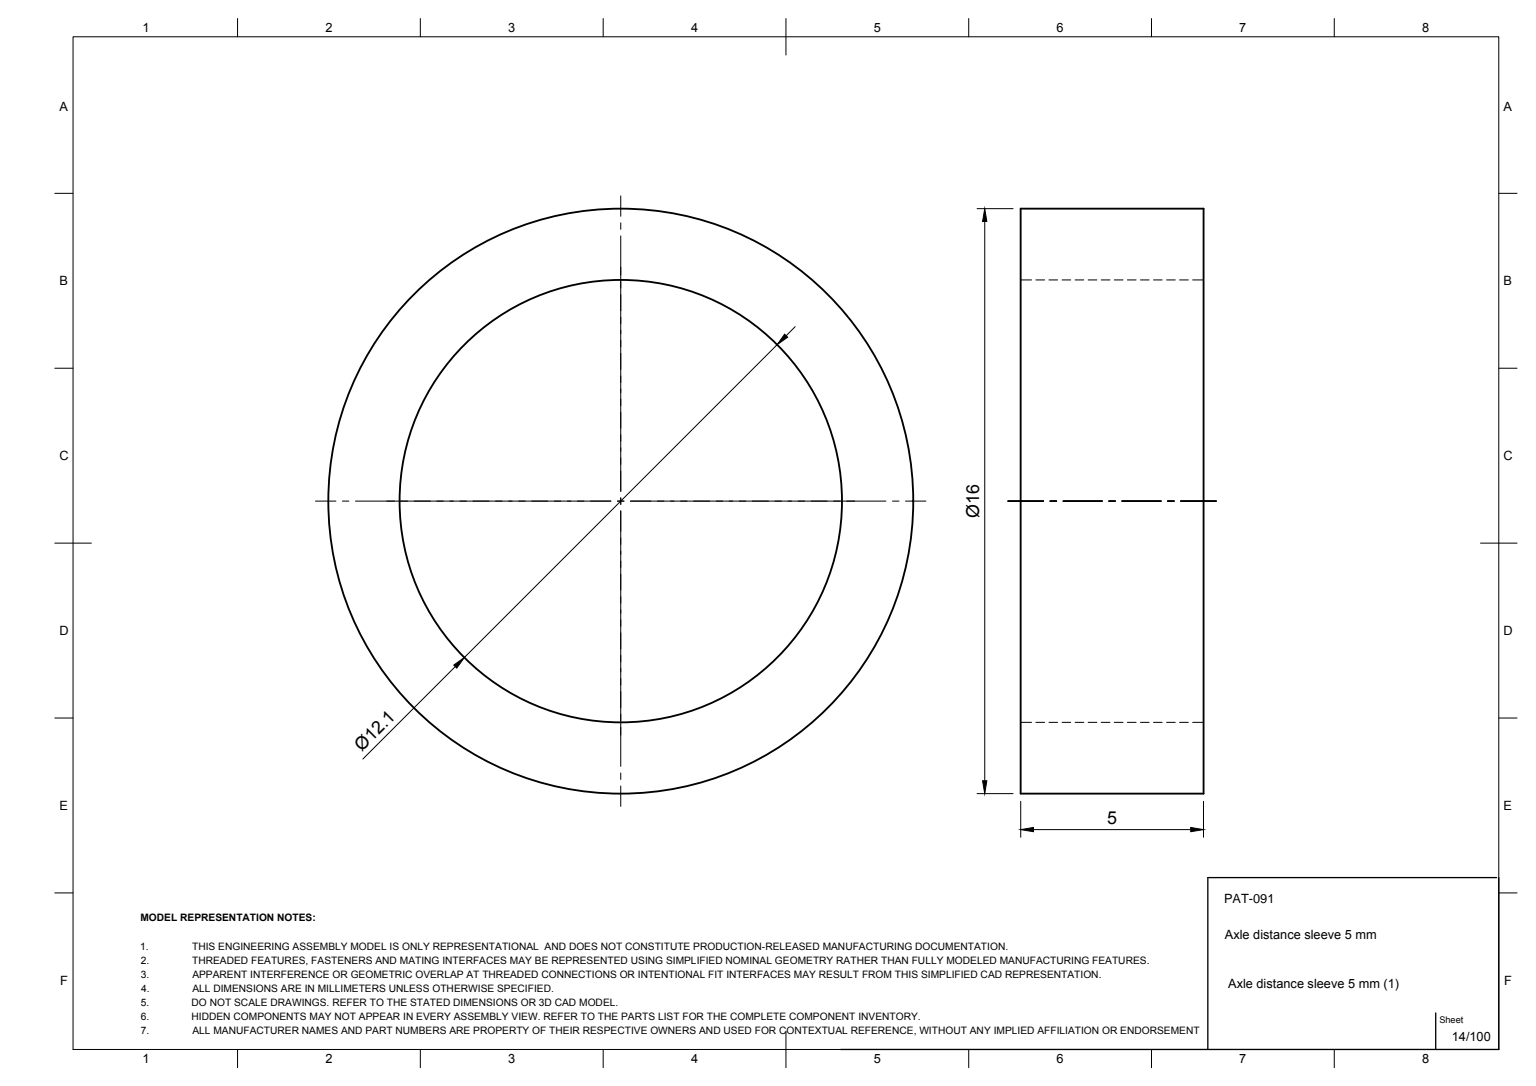
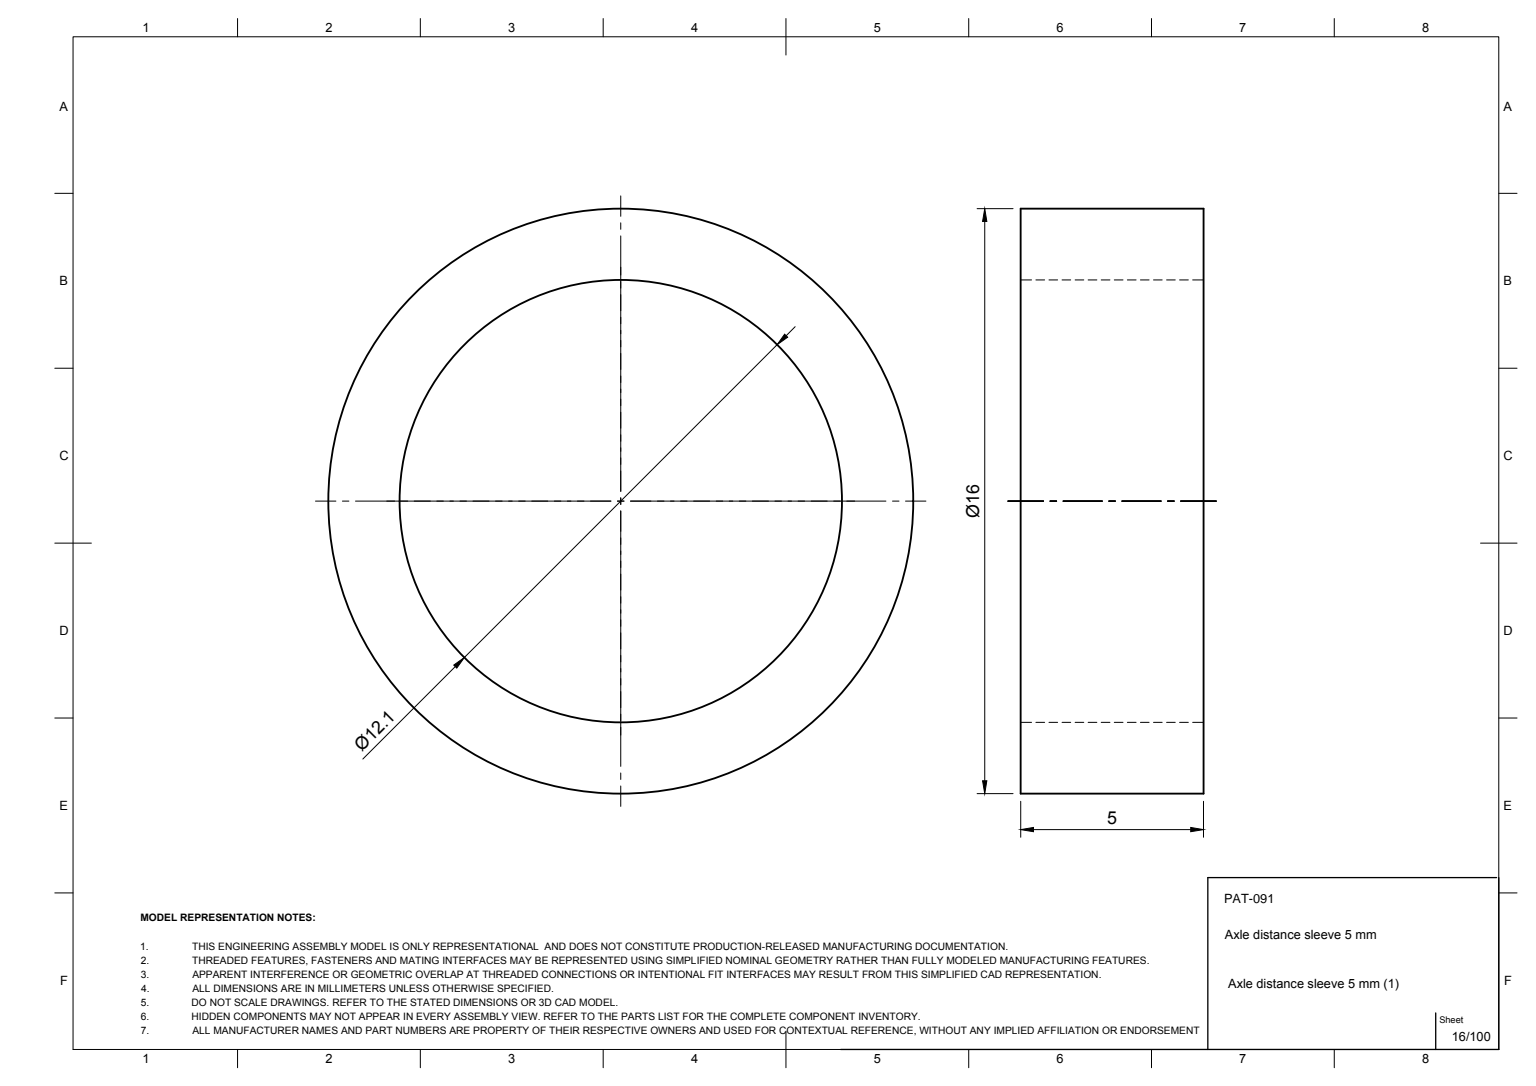
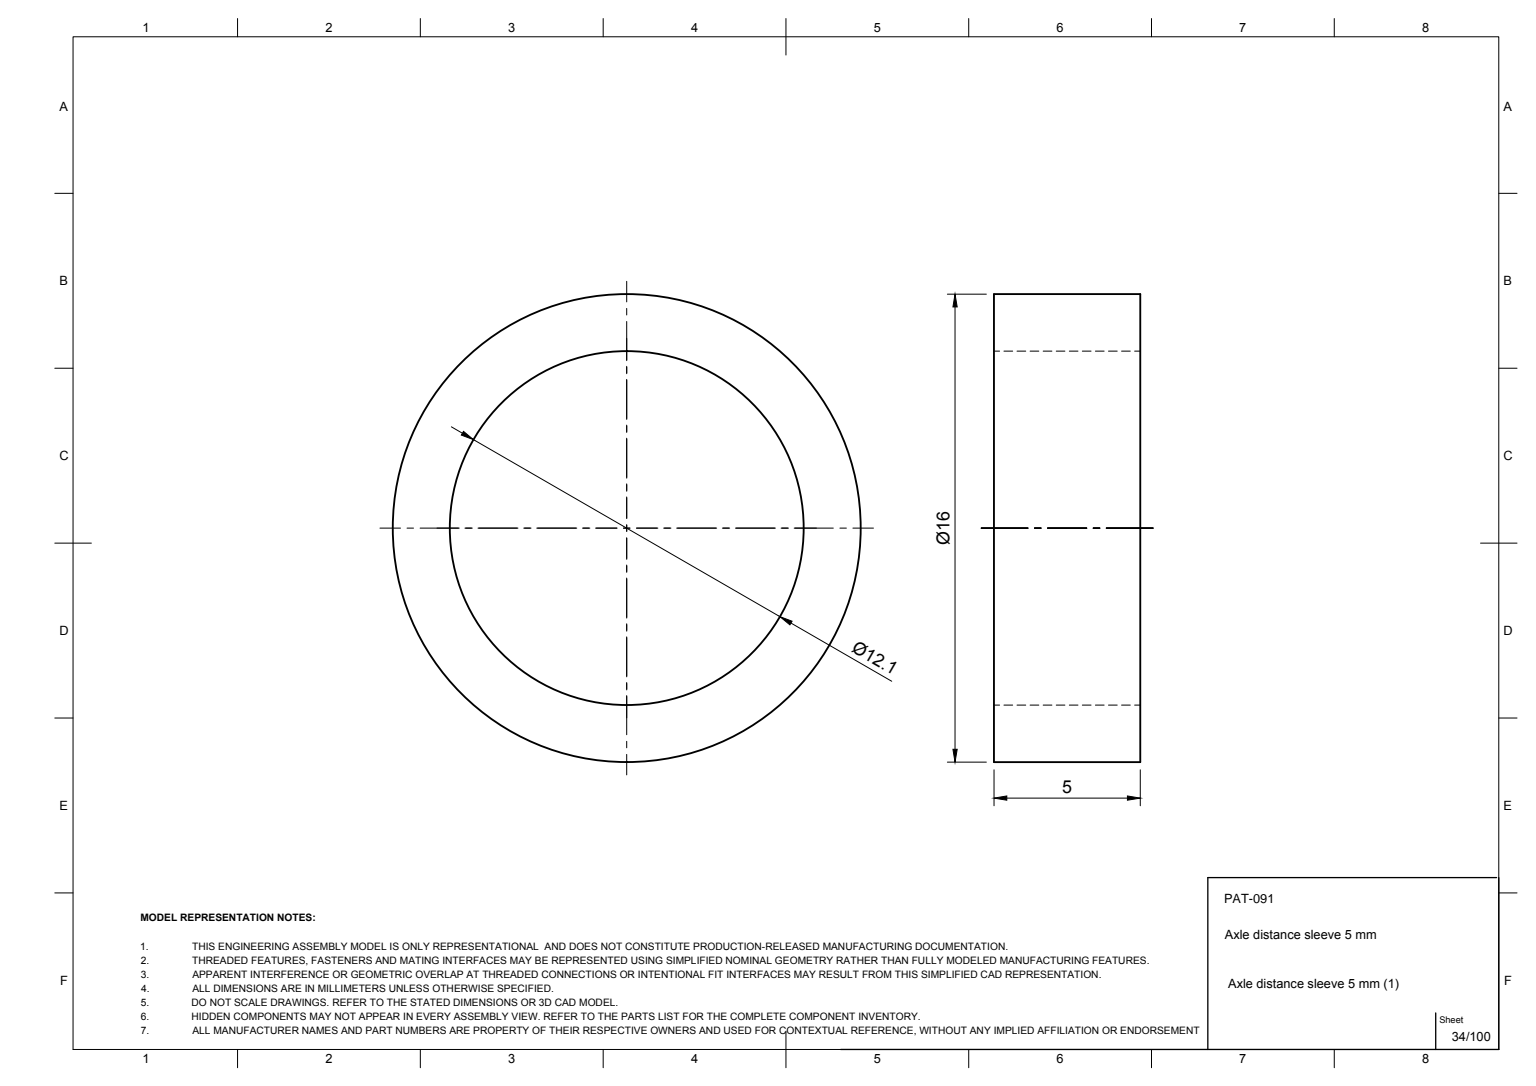
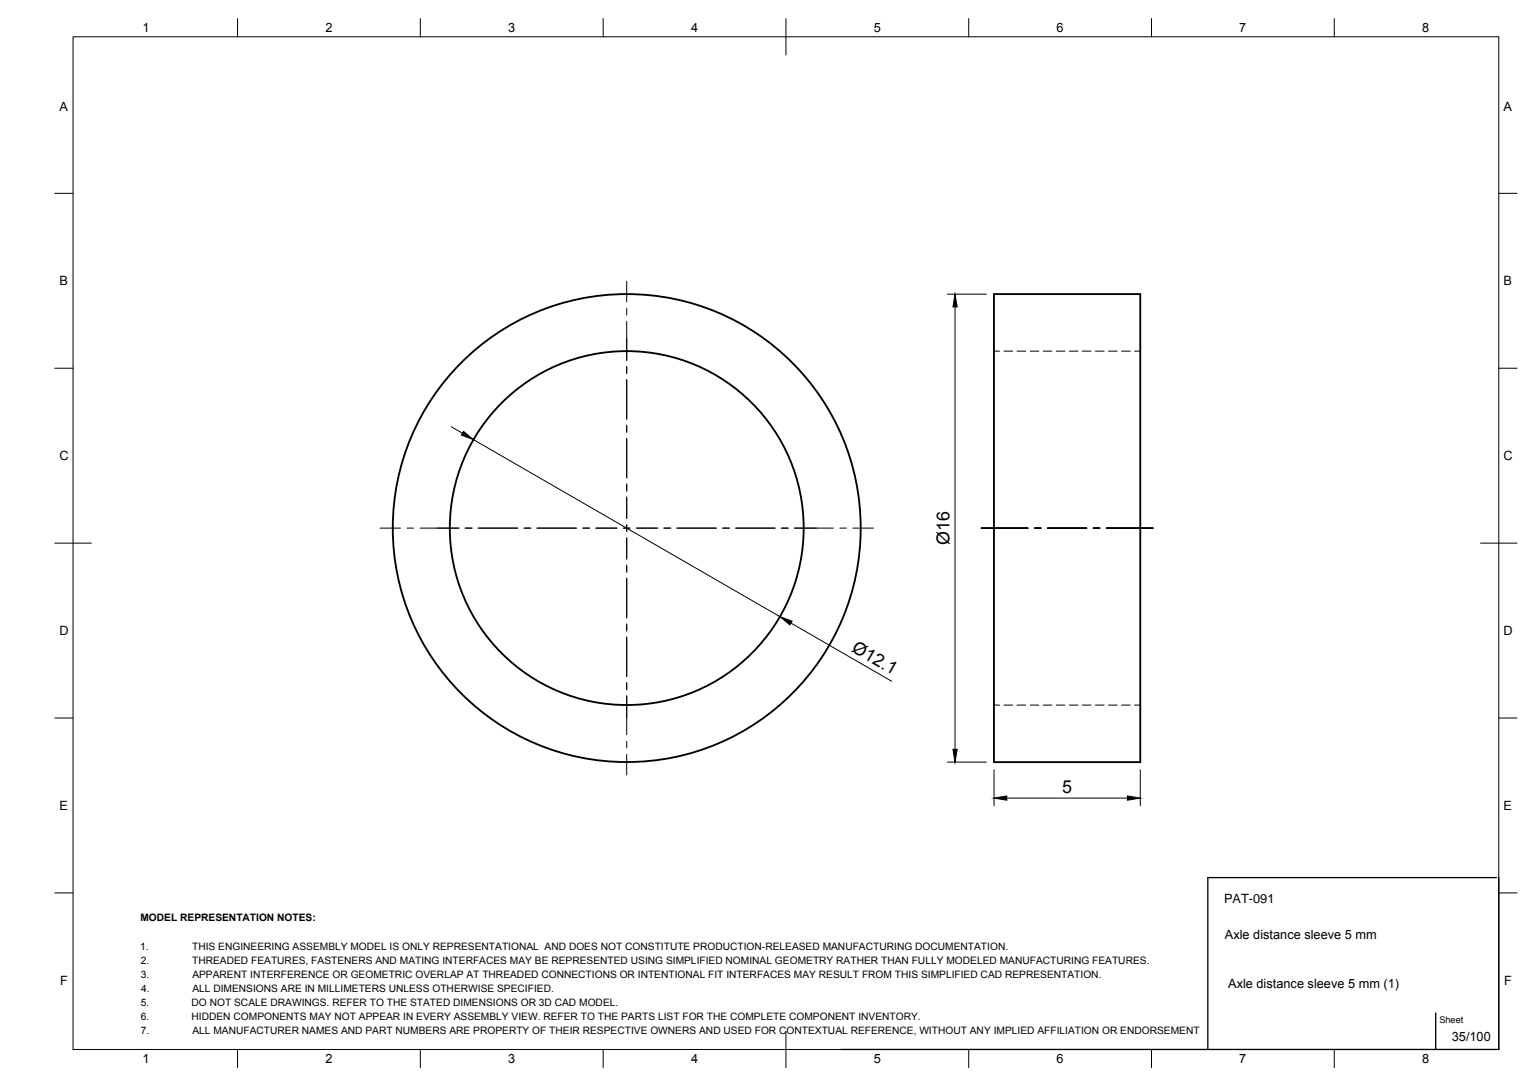
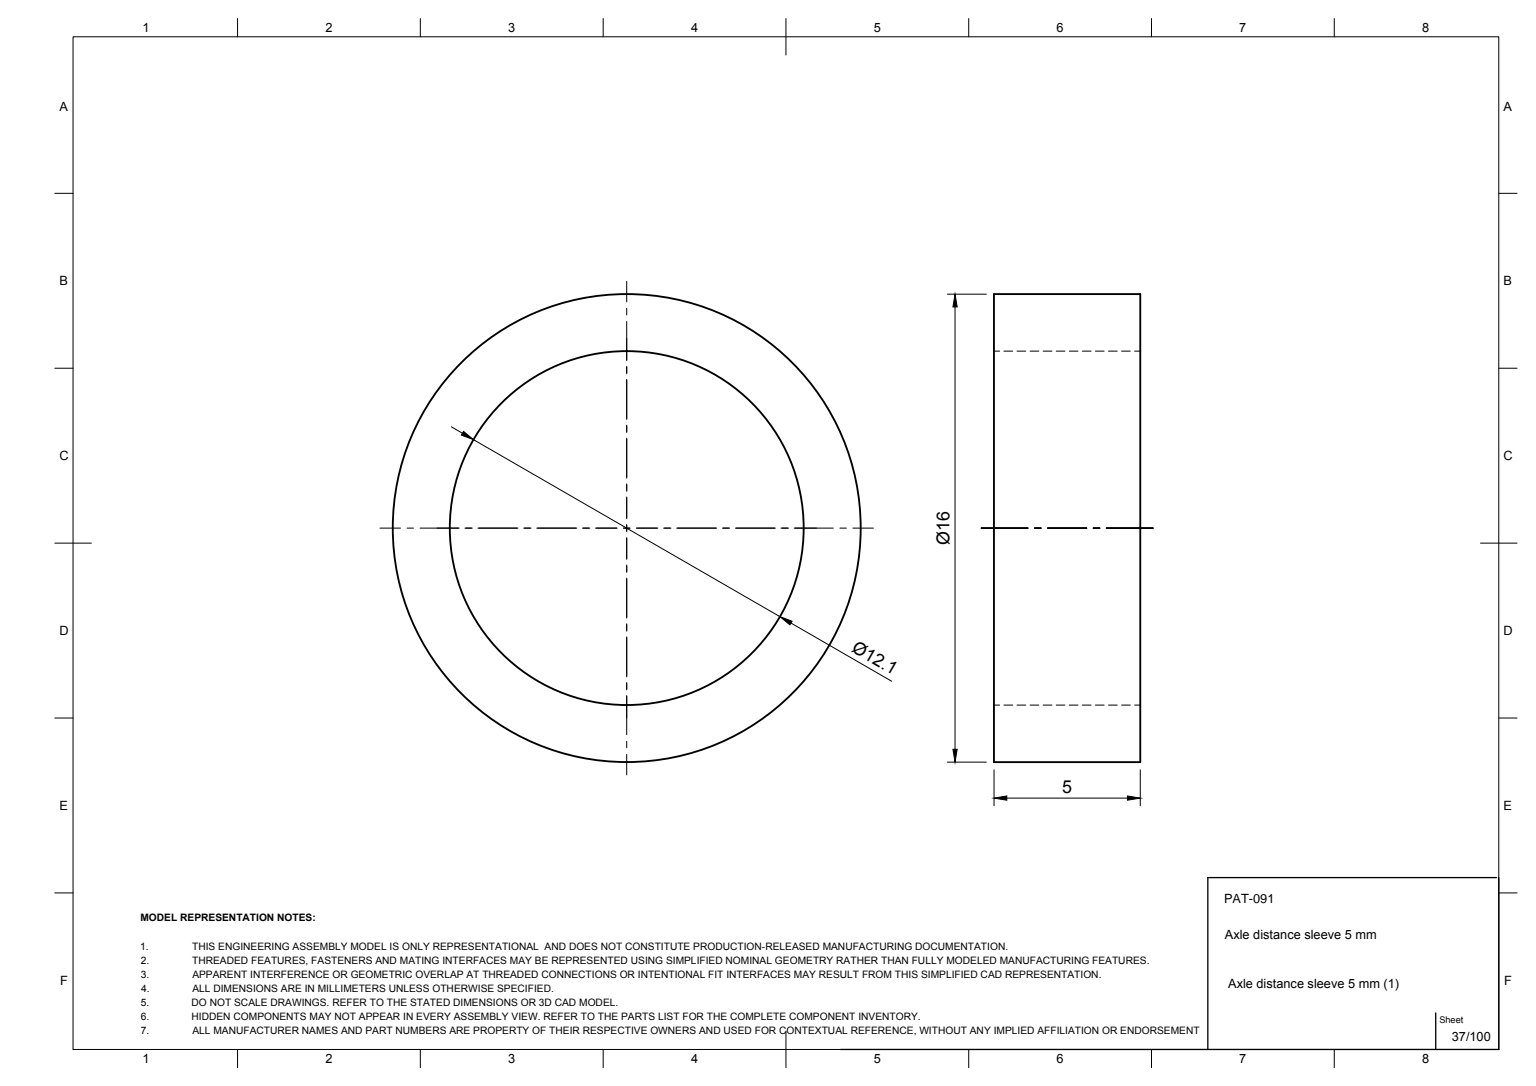
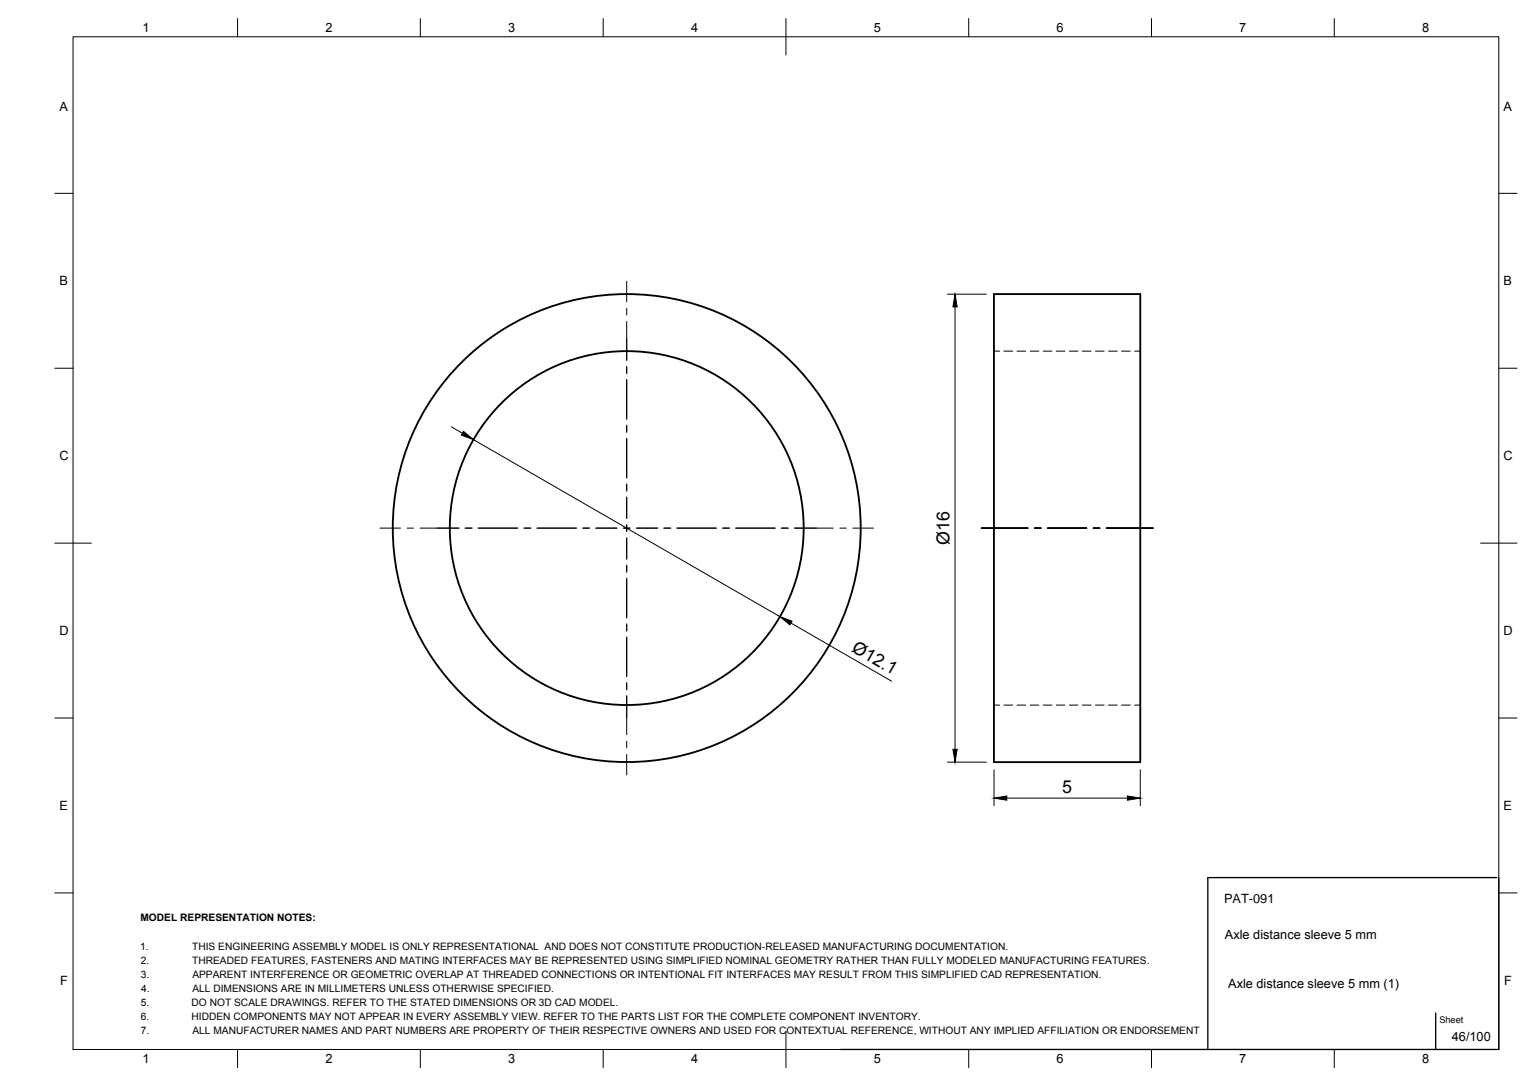
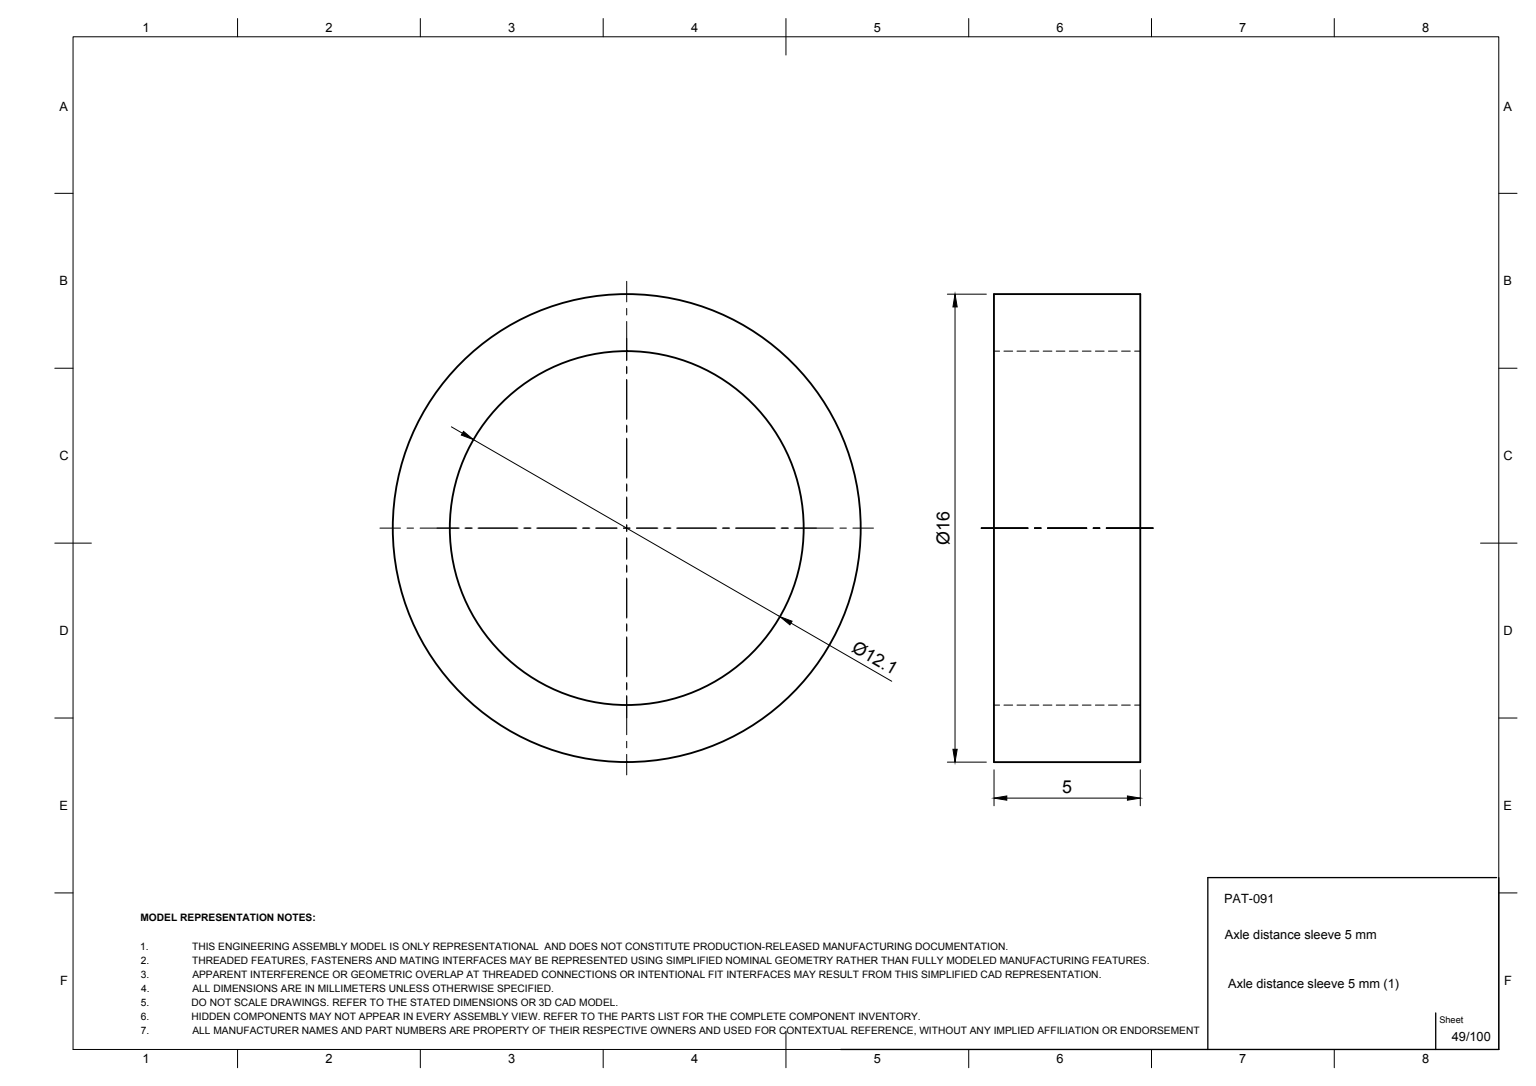
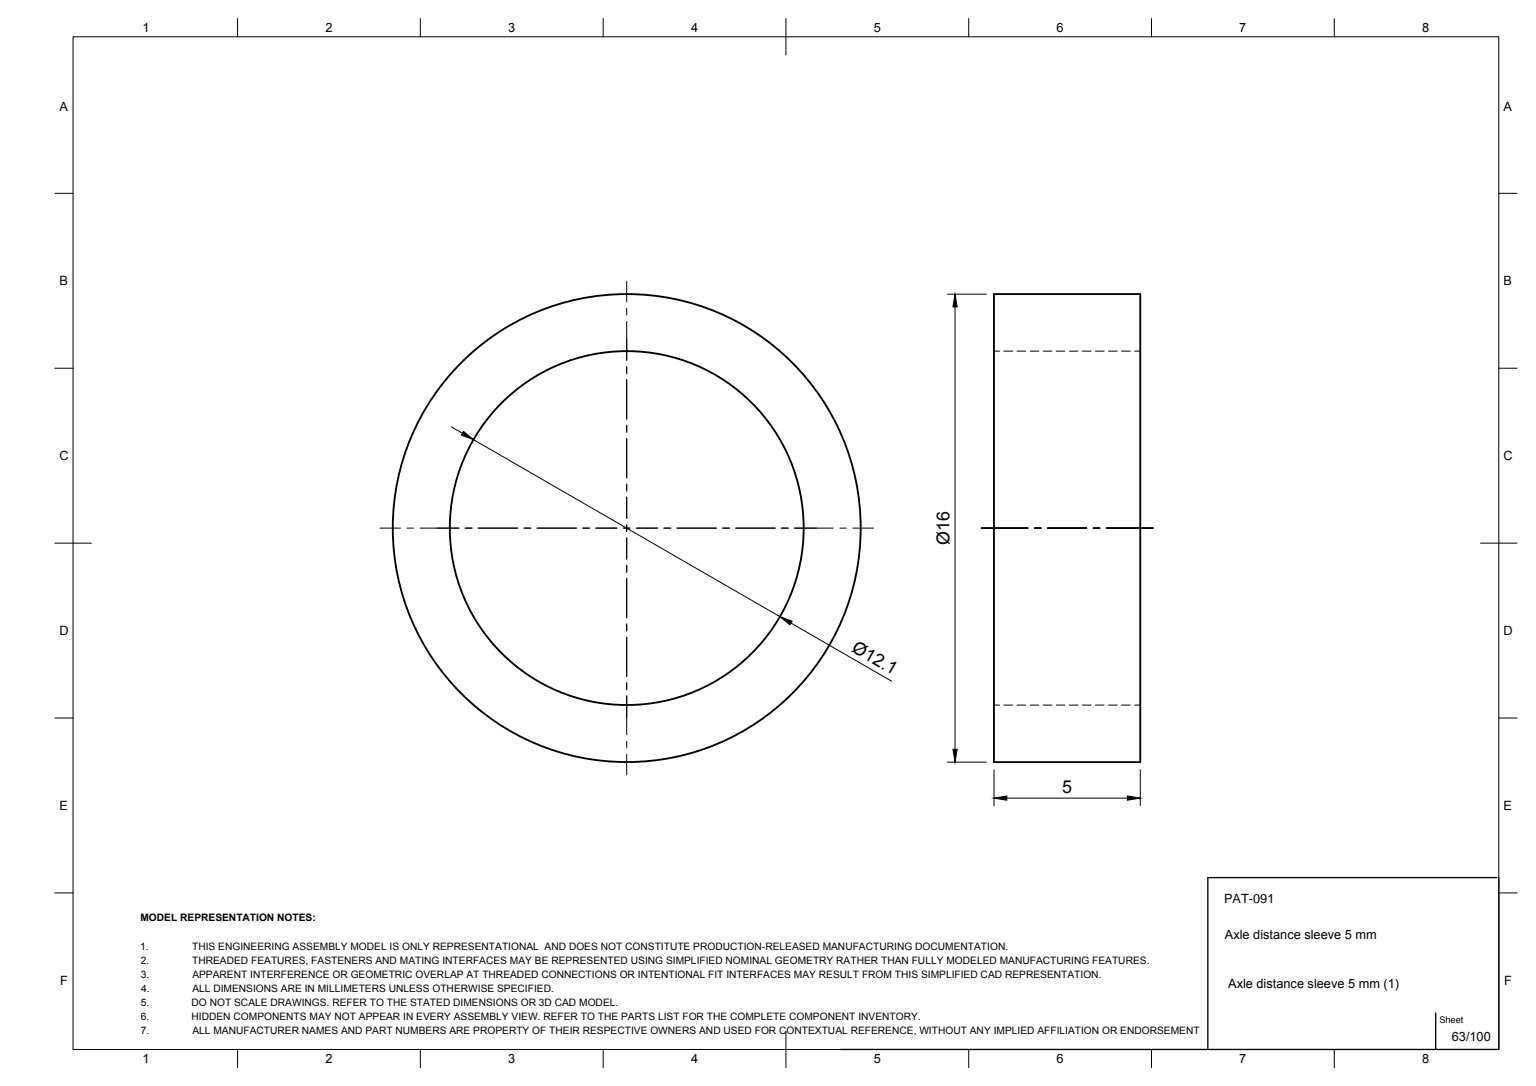
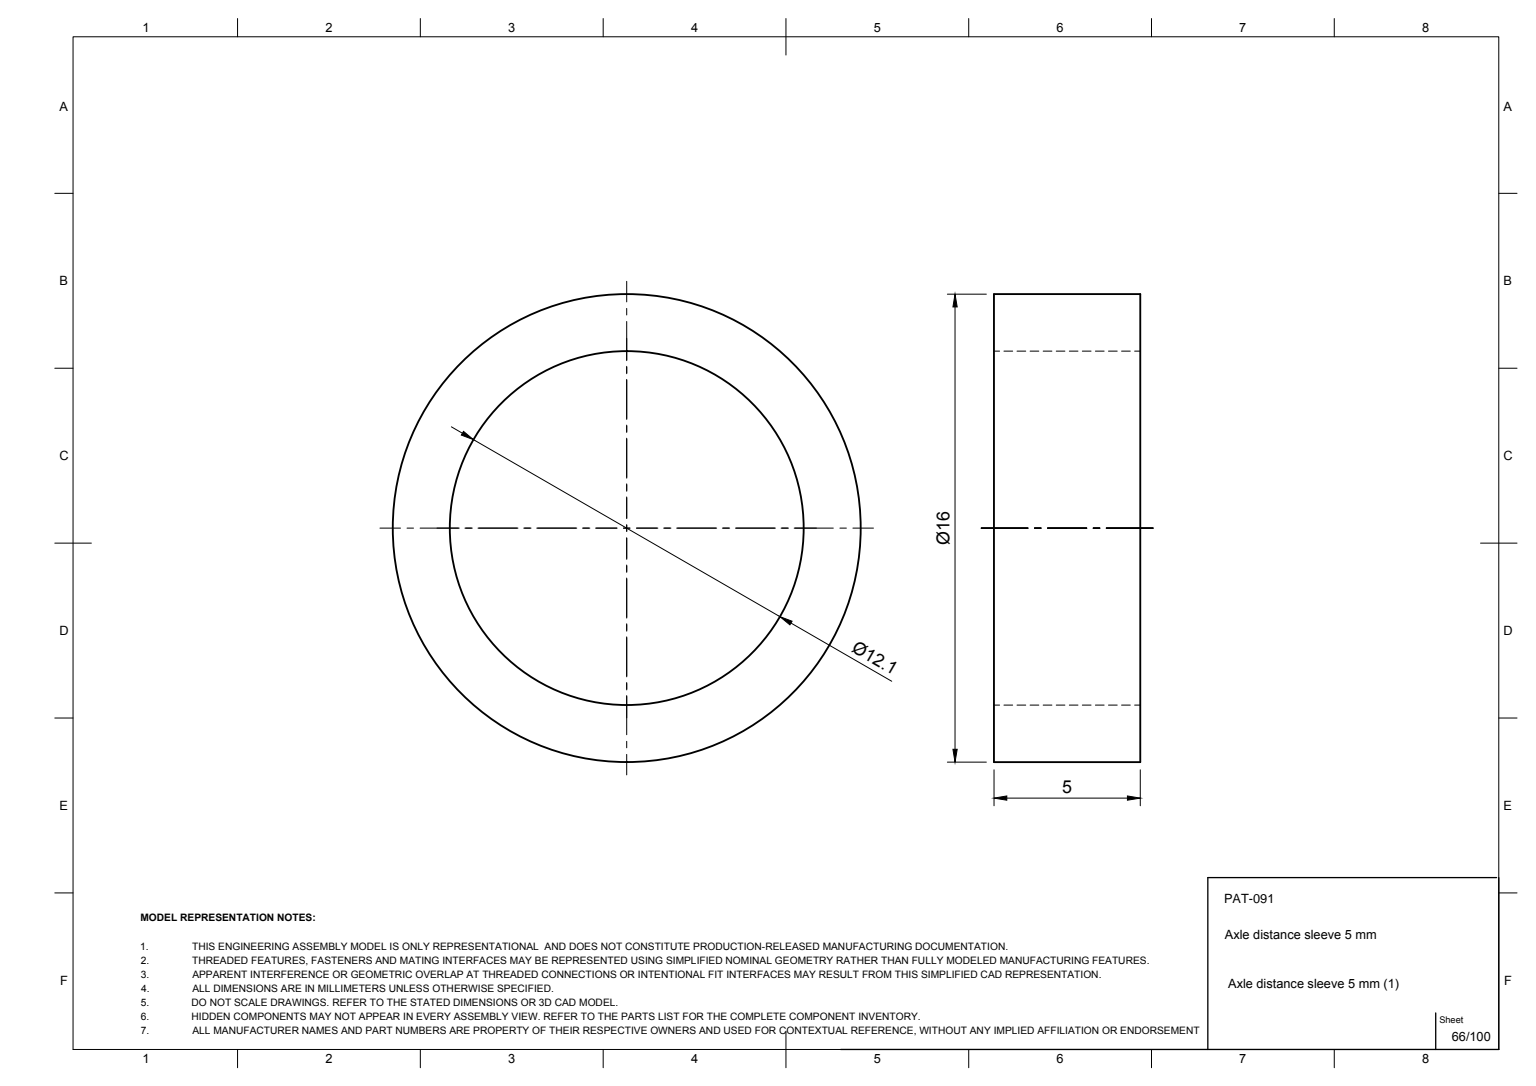
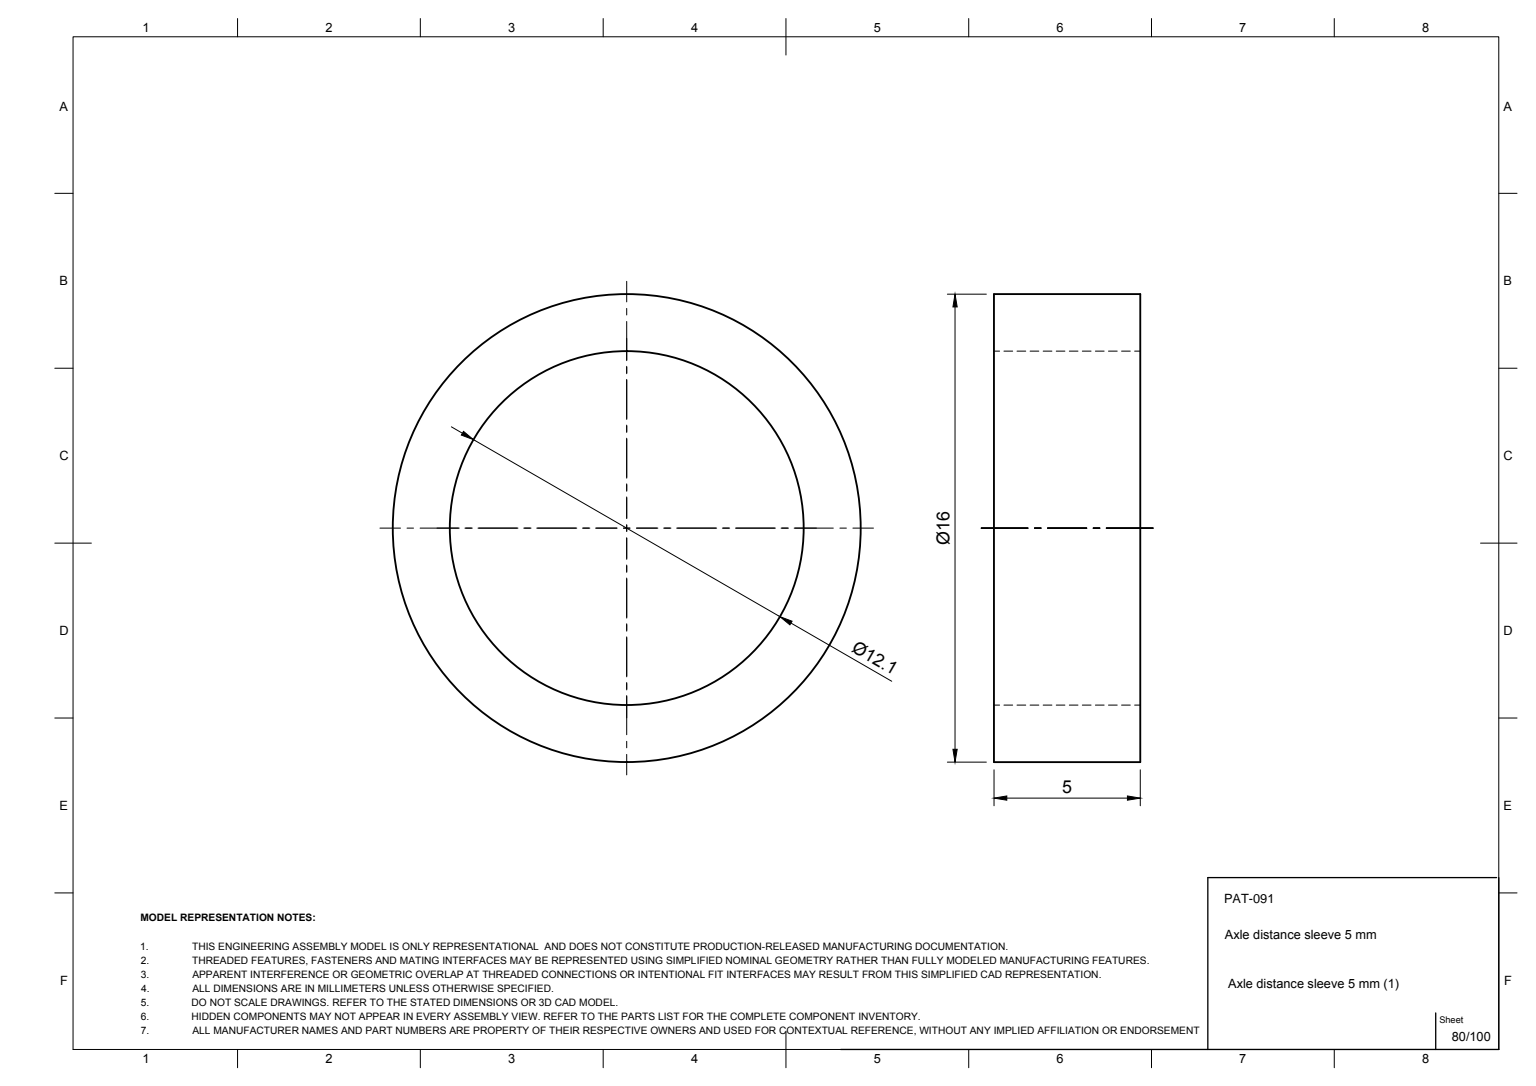
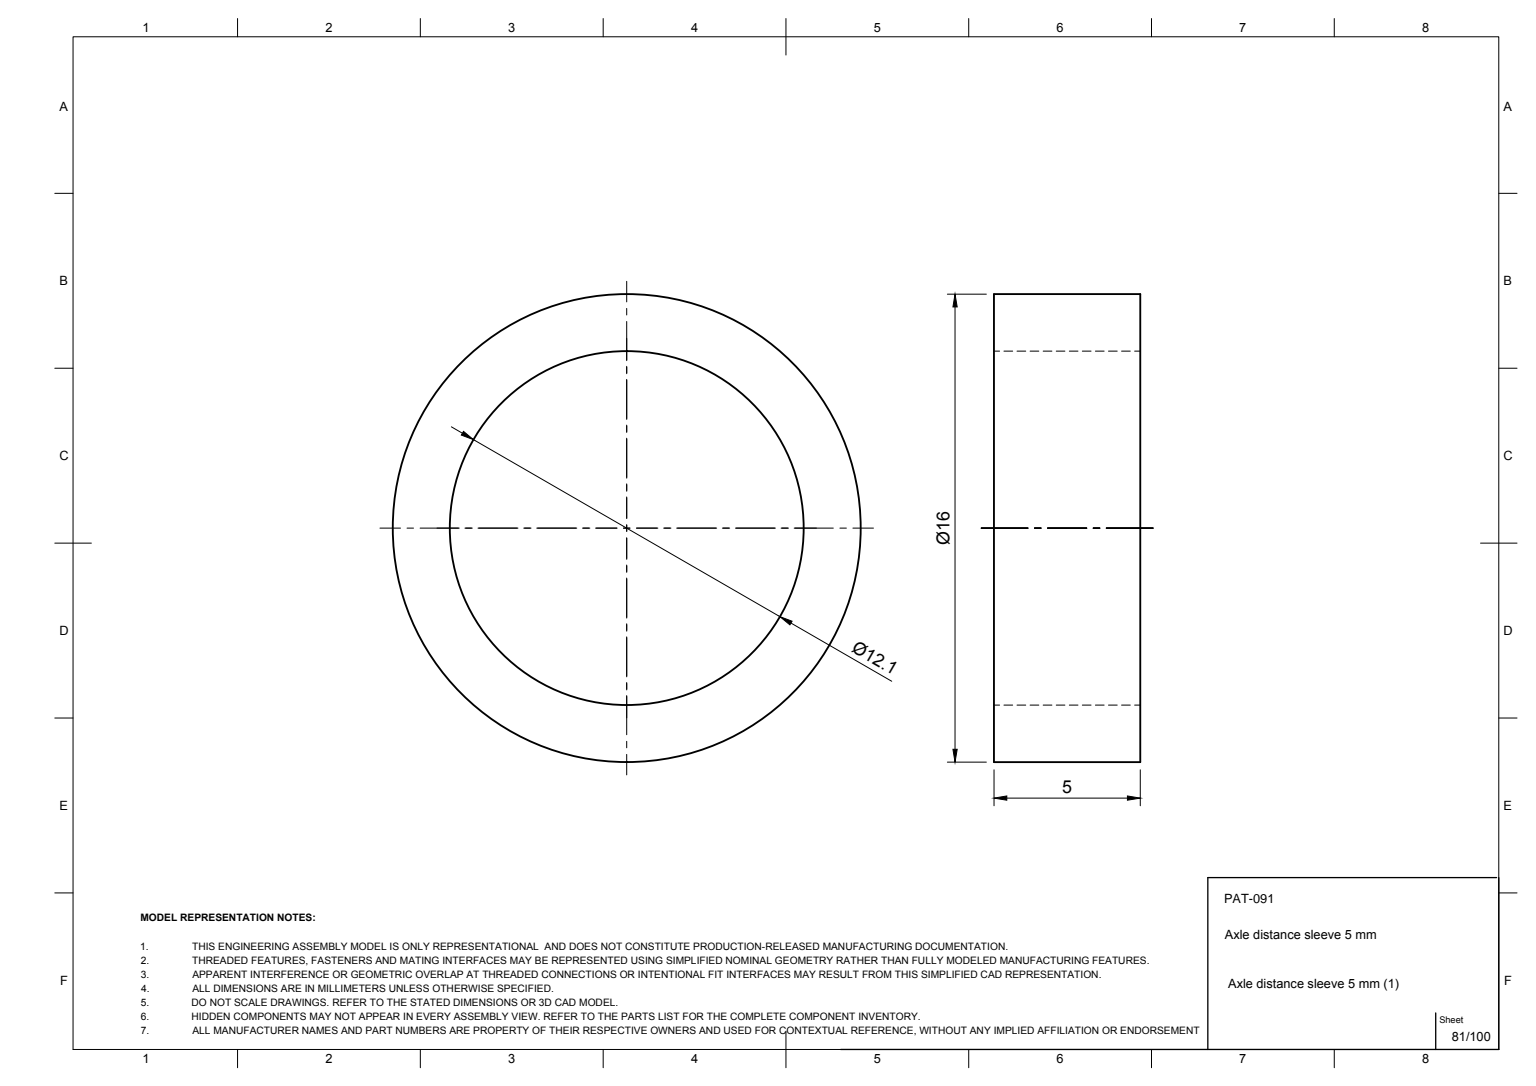
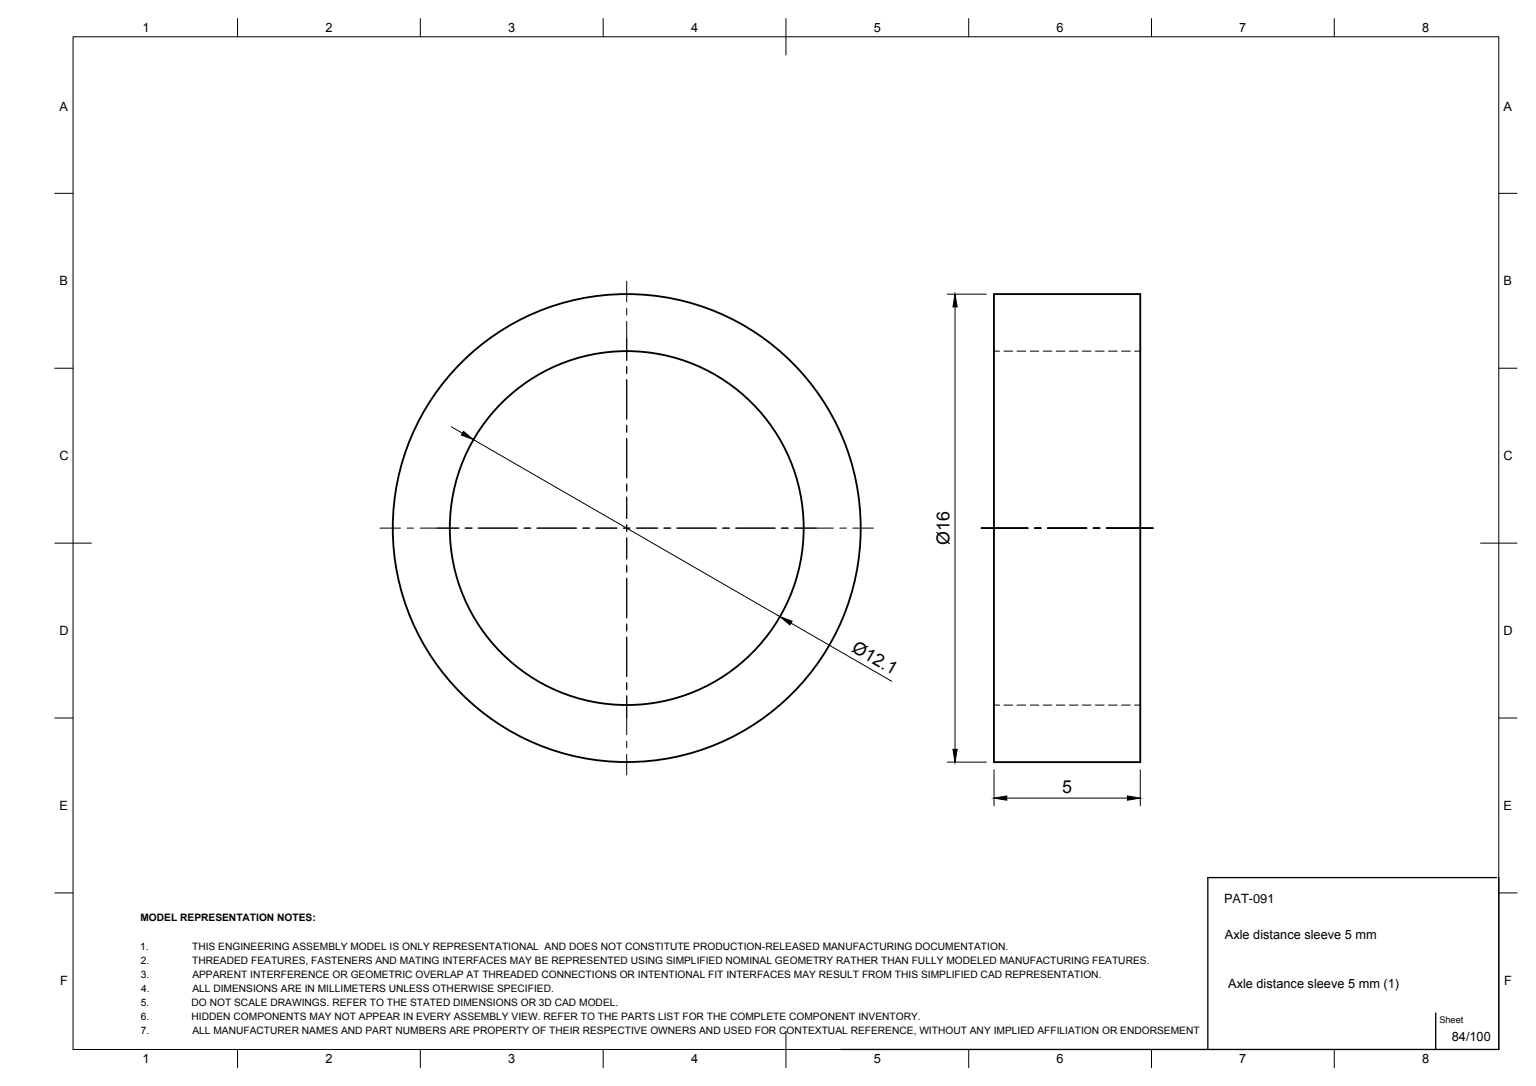
ISO-10303-21;
HEADER;
/* Generated by software containing ST-Developer
 * from STEP Tools, Inc. (www.steptools.com) 
 */

FILE_DESCRIPTION(
/* description */ ('PAT-091'),
/* implementation_level */ '2;1');

FILE_NAME(
/* name */ 'Axle distance sleeve 5 mm.step',
/* time_stamp */ '2026-10-27T15:34:44-07:00',
/* author */ (''),
/* organization */ (''),
/* preprocessor_version */ 'ST-DEVELOPER v20.2',
/* originating_system */ 'Autodesk Translation Framework v15.17.0.0',
/* authorisation */ '');

FILE_SCHEMA (('AUTOMOTIVE_DESIGN { 1 0 10303 214 3 1 1 }'));
ENDSEC;

DATA;
#10=MECHANICAL_DESIGN_GEOMETRIC_PRESENTATION_REPRESENTATION('',(#985),#25100);
#765=SHAPE_REPRESENTATION_RELATIONSHIP('SRR','None',#25526,#875);
#875=ADVANCED_BREP_SHAPE_REPRESENTATION('',(#1109),#24996);
#985=STYLED_ITEM('',(#26191),#1109);
#1109=MANIFOLD_SOLID_BREP('Body1',#13262);
#1327=FACE_BOUND('',#3126,.T.);
#1328=FACE_BOUND('',#3128,.T.);
#1702=PLANE('',#14874);
#1703=PLANE('',#14875);
#2193=FACE_OUTER_BOUND('',#3123,.T.);
#2194=FACE_OUTER_BOUND('',#3124,.T.);
#2195=FACE_OUTER_BOUND('',#3125,.T.);
#2196=FACE_OUTER_BOUND('',#3127,.T.);
#3123=EDGE_LOOP('',(#9548,#9549,#9550,#9551));
#3124=EDGE_LOOP('',(#9552,#9553,#9554,#9555));
#3125=EDGE_LOOP('',(#9556));
#3126=EDGE_LOOP('',(#9557));
#3127=EDGE_LOOP('',(#9558));
#3128=EDGE_LOOP('',(#9559));
#4276=LINE('',#21605,#5016);
#4277=LINE('',#21611,#5017);
#5016=VECTOR('',#17190,0.605);
#5017=VECTOR('',#17197,0.8);
#5740=CIRCLE('',#14869,0.605);
#5741=CIRCLE('',#14870,0.605);
#5742=CIRCLE('',#14872,0.8);
#5743=CIRCLE('',#14873,0.8);
#6575=VERTEX_POINT('',#21602);
#6576=VERTEX_POINT('',#21604);
#6577=VERTEX_POINT('',#21608);
#6578=VERTEX_POINT('',#21610);
#7709=EDGE_CURVE('',#6575,#6575,#5740,.T.);
#7710=EDGE_CURVE('',#6575,#6576,#4276,.T.);
#7711=EDGE_CURVE('',#6576,#6576,#5741,.T.);
#7712=EDGE_CURVE('',#6577,#6577,#5742,.T.);
#7713=EDGE_CURVE('',#6577,#6578,#4277,.T.);
#7714=EDGE_CURVE('',#6578,#6578,#5743,.T.);
#9548=ORIENTED_EDGE('',*,*,#7709,.F.);
#9549=ORIENTED_EDGE('',*,*,#7710,.T.);
#9550=ORIENTED_EDGE('',*,*,#7711,.T.);
#9551=ORIENTED_EDGE('',*,*,#7710,.F.);
#9552=ORIENTED_EDGE('',*,*,#7712,.F.);
#9553=ORIENTED_EDGE('',*,*,#7713,.T.);
#9554=ORIENTED_EDGE('',*,*,#7714,.T.);
#9555=ORIENTED_EDGE('',*,*,#7713,.F.);
#9556=ORIENTED_EDGE('',*,*,#7712,.T.);
#9557=ORIENTED_EDGE('',*,*,#7709,.T.);
#9558=ORIENTED_EDGE('',*,*,#7714,.F.);
#9559=ORIENTED_EDGE('',*,*,#7711,.F.);
#12142=CYLINDRICAL_SURFACE('',#14868,0.605);
#12143=CYLINDRICAL_SURFACE('',#14871,0.8);
#12560=ADVANCED_FACE('',(#2193),#12142,.F.);
#12561=ADVANCED_FACE('',(#2194),#12143,.T.);
#12562=ADVANCED_FACE('',(#2195,#1327),#1702,.T.);
#12563=ADVANCED_FACE('',(#2196,#1328),#1703,.F.);
#13262=CLOSED_SHELL('',(#12560,#12561,#12562,#12563));
#14867=AXIS2_PLACEMENT_3D('',#21600,#17184,#17185);
#14868=AXIS2_PLACEMENT_3D('',#21601,#17186,#17187);
#14869=AXIS2_PLACEMENT_3D('',#21603,#17188,#17189);
#14870=AXIS2_PLACEMENT_3D('',#21606,#17191,#17192);
#14871=AXIS2_PLACEMENT_3D('',#21607,#17193,#17194);
#14872=AXIS2_PLACEMENT_3D('',#21609,#17195,#17196);
#14873=AXIS2_PLACEMENT_3D('',#21612,#17198,#17199);
#14874=AXIS2_PLACEMENT_3D('',#21613,#17200,#17201);
#14875=AXIS2_PLACEMENT_3D('',#21614,#17202,#17203);
#17184=DIRECTION('axis',(0.,0.,1.));
#17185=DIRECTION('refdir',(1.,0.,0.));
#17186=DIRECTION('center_axis',(0.,1.,0.));
#17187=DIRECTION('ref_axis',(1.,0.,0.));
#17188=DIRECTION('center_axis',(0.,-1.,0.));
#17189=DIRECTION('ref_axis',(1.,0.,0.));
#17190=DIRECTION('',(0.,-1.,0.));
#17191=DIRECTION('center_axis',(0.,-1.,0.));
#17192=DIRECTION('ref_axis',(1.,0.,0.));
#17193=DIRECTION('center_axis',(0.,1.,0.));
#17194=DIRECTION('ref_axis',(1.,0.,0.));
#17195=DIRECTION('center_axis',(0.,1.,0.));
#17196=DIRECTION('ref_axis',(1.,0.,0.));
#17197=DIRECTION('',(0.,-1.,0.));
#17198=DIRECTION('center_axis',(0.,1.,0.));
#17199=DIRECTION('ref_axis',(1.,0.,0.));
#17200=DIRECTION('center_axis',(0.,1.,0.));
#17201=DIRECTION('ref_axis',(1.,0.,0.));
#17202=DIRECTION('center_axis',(0.,1.,0.));
#17203=DIRECTION('ref_axis',(1.,0.,0.));
#21600=CARTESIAN_POINT('',(0.,0.,0.));
#21601=CARTESIAN_POINT('Origin',(0.,-7.5,3.));
#21602=CARTESIAN_POINT('',(-0.605,-7.,3.));
#21603=CARTESIAN_POINT('Origin',(0.,-7.,3.));
#21604=CARTESIAN_POINT('',(-0.605,-7.5,3.));
#21605=CARTESIAN_POINT('',(-0.605,-7.5,3.));
#21606=CARTESIAN_POINT('Origin',(0.,-7.5,3.));
#21607=CARTESIAN_POINT('Origin',(0.,-7.5,3.));
#21608=CARTESIAN_POINT('',(-0.8,-7.,3.));
#21609=CARTESIAN_POINT('Origin',(0.,-7.,3.));
#21610=CARTESIAN_POINT('',(-0.8,-7.5,3.));
#21611=CARTESIAN_POINT('',(-0.8,-7.5,3.));
#21612=CARTESIAN_POINT('Origin',(0.,-7.5,3.));
#21613=CARTESIAN_POINT('Origin',(0.,-7.,3.));
#21614=CARTESIAN_POINT('Origin',(0.,-7.5,3.));
#24875=UNCERTAINTY_MEASURE_WITH_UNIT(LENGTH_MEASURE(0.001),#25101,
'DISTANCE_ACCURACY_VALUE',
'Maximum model space distance between geometric entities at asserted c
onnectivities');
#24979=UNCERTAINTY_MEASURE_WITH_UNIT(LENGTH_MEASURE(0.001),#25101,
'DISTANCE_ACCURACY_VALUE',
'Maximum model space distance between geometric entities at asserted c
onnectivities');
#24996=(
GEOMETRIC_REPRESENTATION_CONTEXT(3)
GLOBAL_UNCERTAINTY_ASSIGNED_CONTEXT((#24875))
GLOBAL_UNIT_ASSIGNED_CONTEXT((#25101,#25103,#25104))
REPRESENTATION_CONTEXT('','3D')
);
#25100=(
GEOMETRIC_REPRESENTATION_CONTEXT(3)
GLOBAL_UNCERTAINTY_ASSIGNED_CONTEXT((#24979))
GLOBAL_UNIT_ASSIGNED_CONTEXT((#25101,#25103,#25104))
REPRESENTATION_CONTEXT('','3D')
);
#25101=(
LENGTH_UNIT()
NAMED_UNIT(*)
SI_UNIT(.CENTI.,.METRE.)
);
#25103=(
NAMED_UNIT(*)
PLANE_ANGLE_UNIT()
SI_UNIT($,.RADIAN.)
);
#25104=(
NAMED_UNIT(*)
SI_UNIT($,.STERADIAN.)
SOLID_ANGLE_UNIT()
);
#25121=SHAPE_DEFINITION_REPRESENTATION(#25241,#25526);
#25241=PRODUCT_DEFINITION_SHAPE('',$,#25647);
#25526=SHAPE_REPRESENTATION('',(#14867),#24996);
#25630=PRODUCT_DEFINITION_CONTEXT('part definition',#25992,'design');
#25647=PRODUCT_DEFINITION('Axle distance sleeve 5 mm',
'Axle distance sleeve 5 mm',#25767,#25630);
#25767=PRODUCT_DEFINITION_FORMATION('',$,#26010);
#25992=APPLICATION_CONTEXT(
'Core Data for Automotive Mechanical Design Process');
#25993=PRODUCT_CONTEXT('part definition',#25992,'mechanical');
#26010=PRODUCT('Axle distance sleeve 5 mm','Axle distance sleeve 5 mm',
'Axle distance sleeve 5 mm',(#25993));
#26185=COLOUR_RGB('Grey',0.48,0.52,0.57);
#26186=FILL_AREA_STYLE_COLOUR('',#26185);
#26187=FILL_AREA_STYLE('',(#26186));
#26188=SURFACE_STYLE_FILL_AREA(#26187);
#26189=SURFACE_SIDE_STYLE('',(#26188));
#26190=SURFACE_STYLE_USAGE(.BOTH.,#26189);
#26191=PRESENTATION_STYLE_ASSIGNMENT((#26190));
ENDSEC;
END-ISO-10303-21;
